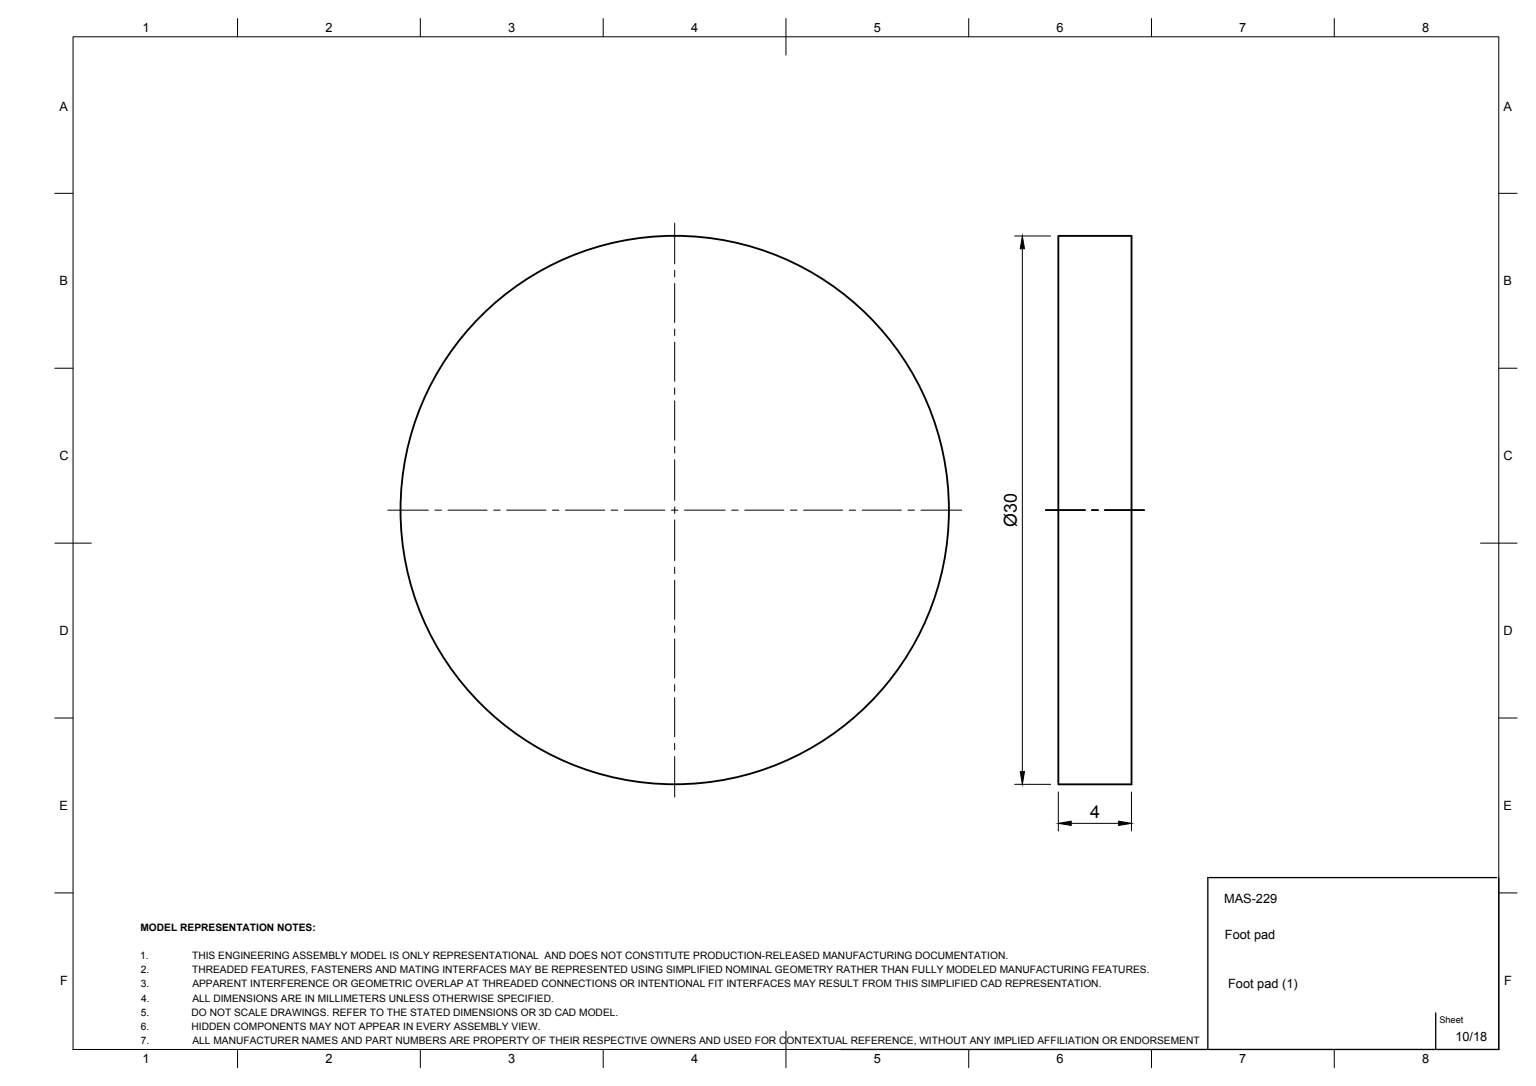
ISO-10303-21;
HEADER;
/* Generated by software containing ST-Developer
 * from STEP Tools, Inc. (www.steptools.com) 
 */

FILE_DESCRIPTION(
/* description */ ('Independently dimensioned six-bar single-leg walking-linkage demonstr
ator. Whole-mm20 crank,60 upper rocker,80/120 ternary coupler,120 lowe
r rocker,140 knee pitch and260 toe reach; ground pivots0/0,60/0,40/60.
 Seven native revolutes close both loops. Four reused native library f
amilies, fully retained shared pins and layered real spacer stacks, bo
nded rubber toe. Benchtop reference mechanism; no complete vehicle, lo
ad, gait stability, adhesive, weld, fit or life rating.'),
/* implementation_level */ '2;1');

FILE_NAME(
/* name */ 'Foot pad.step',
/* time_stamp */ '2026-11-09T20:33:14-08:00',
/* author */ (''),
/* organization */ (''),
/* preprocessor_version */ 'ST-DEVELOPER v20.2',
/* originating_system */ 'Autodesk Translation Framework v15.17.0.0',
/* authorisation */ '');

FILE_SCHEMA (('AUTOMOTIVE_DESIGN { 1 0 10303 214 3 1 1 }'));
ENDSEC;

DATA;
#10=MECHANICAL_DESIGN_GEOMETRIC_PRESENTATION_REPRESENTATION('',(#262),#4048);
#226=SHAPE_REPRESENTATION_RELATIONSHIP('SRR','None',#4150,#244);
#244=ADVANCED_BREP_SHAPE_REPRESENTATION('',(#280),#4037);
#262=STYLED_ITEM('',(#4249),#280);
#280=MANIFOLD_SOLID_BREP('Body1',#2151);
#382=PLANE('',#2491);
#383=PLANE('',#2492);
#477=FACE_OUTER_BOUND('',#639,.T.);
#478=FACE_OUTER_BOUND('',#640,.T.);
#479=FACE_OUTER_BOUND('',#641,.T.);
#639=EDGE_LOOP('',(#1773,#1774,#1775,#1776));
#640=EDGE_LOOP('',(#1777));
#641=EDGE_LOOP('',(#1778));
#812=LINE('',#3731,#937);
#937=VECTOR('',#3017,15.);
#1030=CIRCLE('',#2489,15.);
#1031=CIRCLE('',#2490,15.);
#1184=VERTEX_POINT('',#3728);
#1185=VERTEX_POINT('',#3730);
#1390=EDGE_CURVE('',#1184,#1184,#1030,.T.);
#1391=EDGE_CURVE('',#1184,#1185,#812,.T.);
#1392=EDGE_CURVE('',#1185,#1185,#1031,.T.);
#1773=ORIENTED_EDGE('',*,*,#1390,.F.);
#1774=ORIENTED_EDGE('',*,*,#1391,.T.);
#1775=ORIENTED_EDGE('',*,*,#1392,.T.);
#1776=ORIENTED_EDGE('',*,*,#1391,.F.);
#1777=ORIENTED_EDGE('',*,*,#1390,.T.);
#1778=ORIENTED_EDGE('',*,*,#1392,.F.);
#1991=CYLINDRICAL_SURFACE('',#2488,15.);
#2080=ADVANCED_FACE('',(#477),#1991,.T.);
#2081=ADVANCED_FACE('',(#478),#382,.T.);
#2082=ADVANCED_FACE('',(#479),#383,.F.);
#2151=CLOSED_SHELL('',(#2080,#2081,#2082));
#2487=AXIS2_PLACEMENT_3D('',#3726,#3011,#3012);
#2488=AXIS2_PLACEMENT_3D('',#3727,#3013,#3014);
#2489=AXIS2_PLACEMENT_3D('',#3729,#3015,#3016);
#2490=AXIS2_PLACEMENT_3D('',#3732,#3018,#3019);
#2491=AXIS2_PLACEMENT_3D('',#3733,#3020,#3021);
#2492=AXIS2_PLACEMENT_3D('',#3734,#3022,#3023);
#3011=DIRECTION('axis',(0.,0.,1.));
#3012=DIRECTION('refdir',(1.,0.,0.));
#3013=DIRECTION('center_axis',(0.,0.,1.));
#3014=DIRECTION('ref_axis',(1.,0.,0.));
#3015=DIRECTION('center_axis',(0.,0.,1.));
#3016=DIRECTION('ref_axis',(1.,0.,0.));
#3017=DIRECTION('',(0.,0.,-1.));
#3018=DIRECTION('center_axis',(0.,0.,1.));
#3019=DIRECTION('ref_axis',(1.,0.,0.));
#3020=DIRECTION('center_axis',(0.,0.,1.));
#3021=DIRECTION('ref_axis',(1.,0.,0.));
#3022=DIRECTION('center_axis',(0.,0.,1.));
#3023=DIRECTION('ref_axis',(1.,0.,0.));
#3726=CARTESIAN_POINT('',(0.,0.,0.));
#3727=CARTESIAN_POINT('Origin',(0.,0.,0.));
#3728=CARTESIAN_POINT('',(-15.,-1.83697019872103E-15,4.));
#3729=CARTESIAN_POINT('Origin',(0.,0.,4.));
#3730=CARTESIAN_POINT('',(-15.,-1.83697019872103E-15,0.));
#3731=CARTESIAN_POINT('',(-15.,-1.83697019872103E-15,0.));
#3732=CARTESIAN_POINT('Origin',(0.,0.,0.));
#3733=CARTESIAN_POINT('Origin',(0.,0.,4.));
#3734=CARTESIAN_POINT('Origin',(0.,0.,0.));
#4017=UNCERTAINTY_MEASURE_WITH_UNIT(LENGTH_MEASURE(0.01),#4049,
'DISTANCE_ACCURACY_VALUE',
'Maximum model space distance between geometric entities at asserted c
onnectivities');
#4028=UNCERTAINTY_MEASURE_WITH_UNIT(LENGTH_MEASURE(0.01),#4049,
'DISTANCE_ACCURACY_VALUE',
'Maximum model space distance between geometric entities at asserted c
onnectivities');
#4037=(
GEOMETRIC_REPRESENTATION_CONTEXT(3)
GLOBAL_UNCERTAINTY_ASSIGNED_CONTEXT((#4017))
GLOBAL_UNIT_ASSIGNED_CONTEXT((#4049,#4051,#4052))
REPRESENTATION_CONTEXT('','3D')
);
#4048=(
GEOMETRIC_REPRESENTATION_CONTEXT(3)
GLOBAL_UNCERTAINTY_ASSIGNED_CONTEXT((#4028))
GLOBAL_UNIT_ASSIGNED_CONTEXT((#4049,#4051,#4052))
REPRESENTATION_CONTEXT('','3D')
);
#4049=(
LENGTH_UNIT()
NAMED_UNIT(*)
SI_UNIT(.MILLI.,.METRE.)
);
#4051=(
NAMED_UNIT(*)
PLANE_ANGLE_UNIT()
SI_UNIT($,.RADIAN.)
);
#4052=(
NAMED_UNIT(*)
SI_UNIT($,.STERADIAN.)
SOLID_ANGLE_UNIT()
);
#4061=SHAPE_DEFINITION_REPRESENTATION(#4080,#4150);
#4080=PRODUCT_DEFINITION_SHAPE('',$,#4170);
#4150=SHAPE_REPRESENTATION('',(#2487),#4037);
#4161=PRODUCT_DEFINITION_CONTEXT('part definition',#4220,'design');
#4170=PRODUCT_DEFINITION('Foot pad','Foot pad',#4189,#4161);
#4189=PRODUCT_DEFINITION_FORMATION('',$,#4230);
#4220=APPLICATION_CONTEXT(
'Core Data for Automotive Mechanical Design Process');
#4221=PRODUCT_CONTEXT('part definition',#4220,'mechanical');
#4230=PRODUCT('Foot pad','Foot pad','Foot pad',(#4221));
#4249=PRESENTATION_STYLE_ASSIGNMENT((#4263));
#4263=SURFACE_STYLE_USAGE(.BOTH.,#4277);
#4277=SURFACE_SIDE_STYLE('',(#4291));
#4291=SURFACE_STYLE_FILL_AREA(#4305);
#4305=FILL_AREA_STYLE('Foot charcoal',(#4319));
#4319=FILL_AREA_STYLE_COLOUR('Foot charcoal',#4333);
#4333=COLOUR_RGB('Foot charcoal',0.164705882352941,0.184313725490196,0.211764705882353);
ENDSEC;
END-ISO-10303-21;
